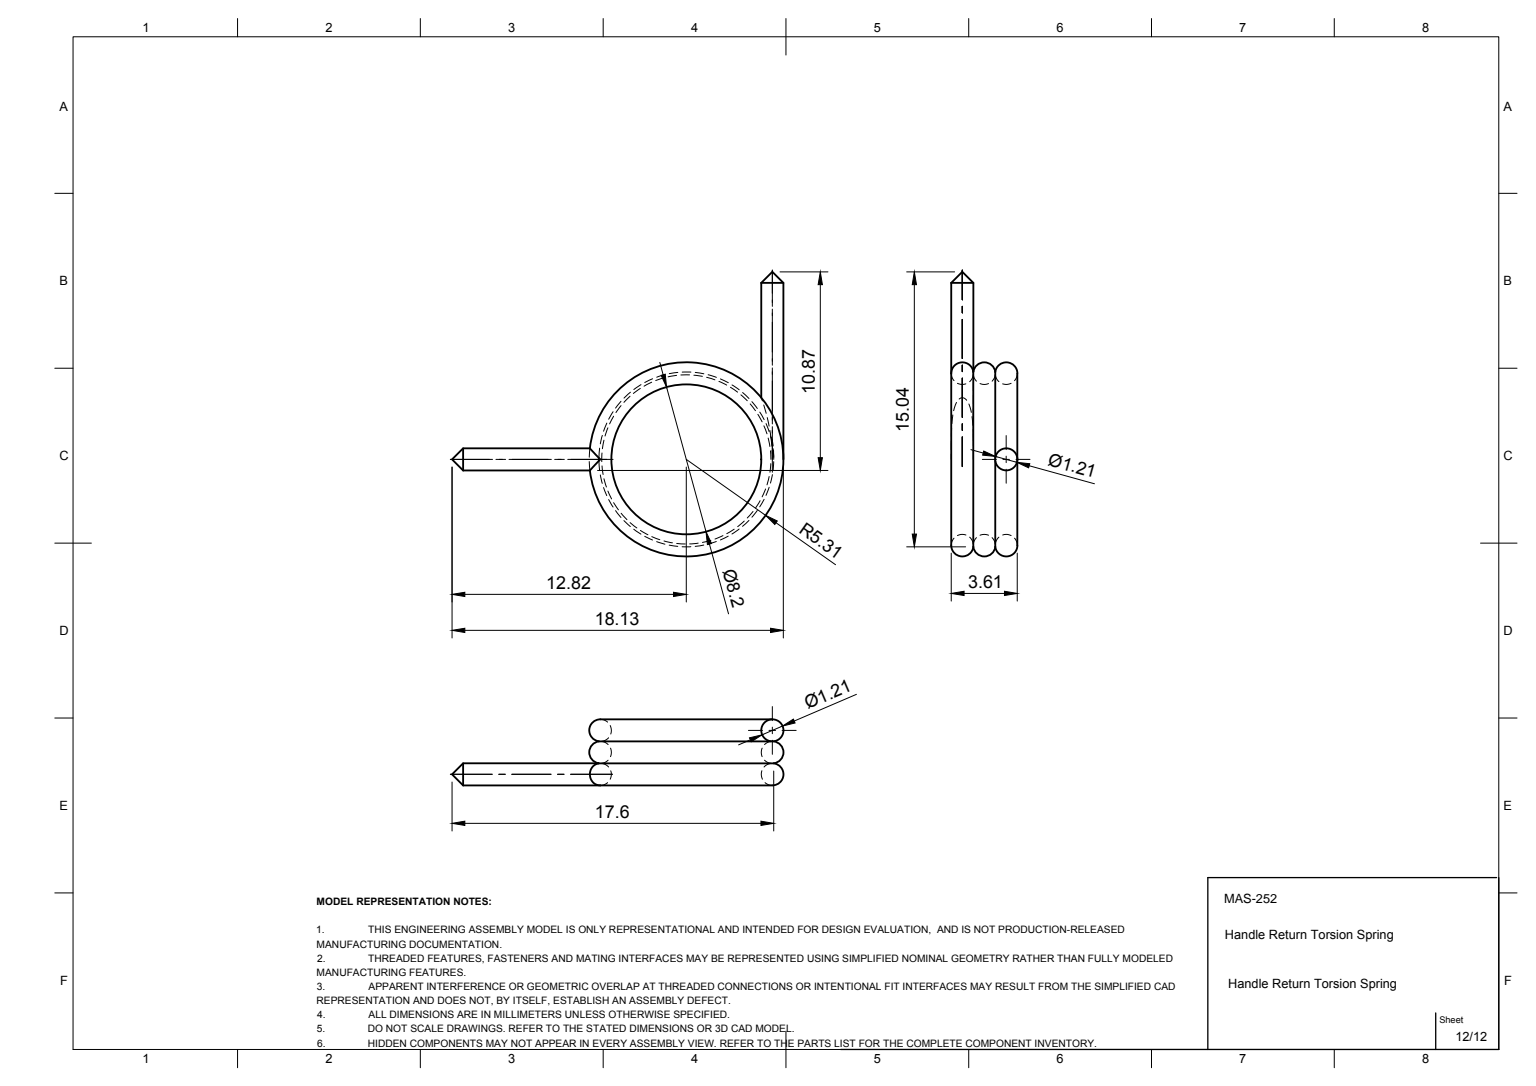
ISO-10303-21;
HEADER;
FILE_DESCRIPTION((''),'2;1');
FILE_NAME('Handle Return Torsion Spring.step','2026-10-06T07:01:46+05:00',(''),(''),'','','');
FILE_SCHEMA (('AUTOMOTIVE_DESIGN { 1 0 10303 214 3 1 1 }'));
ENDSEC;
DATA;
#10=MECHANICAL_DESIGN_GEOMETRIC_PRESENTATION_REPRESENTATION('',(#146),#11396);
#104=CONICAL_SURFACE('',#6292,0.605,0.785398163397447) ;
#105=CONICAL_SURFACE('',#6305,0.605,0.78539816339745) ;
#116=SHAPE_REPRESENTATION_RELATIONSHIP('SRR','None',#11463,#131) ;
#131=ADVANCED_BREP_SHAPE_REPRESENTATION('',(#161),#11389) ;
#146=STYLED_ITEM('',(#11547),#161) ;
#161=MANIFOLD_SOLID_BREP('Handle Return Torsion Spring',#5577) ;
#234=TOROIDAL_SURFACE('',#6293,4.705,0.605) ;
#235=TOROIDAL_SURFACE('',#6298,4.705,0.605) ;
#236=TOROIDAL_SURFACE('',#6306,4.705,0.605) ;
#237=TOROIDAL_SURFACE('',#6309,4.705,0.605) ;
#331=B_SPLINE_CURVE_WITH_KNOTS('',3,(#10992,#10993,#10994,#10995,#10996,
#10997,#10998,#10999,#11000,#11001,#11002,#11003,#11004,#11005),
 .UNSPECIFIED.,.F.,.F.,(4,2,2,2,2,2,4),(-0.0259307736234173,-0.0249485644999998,
-0.0216439933226257,-0.0192686778677155,-0.0180929024728077,-0.0172645332734243,
-0.0172587275311834),.UNSPECIFIED.) ;
#332=B_SPLINE_CURVE_WITH_KNOTS('',3,(#11007,#11008,#11009,#11010,#11011,
#11012,#11013,#11014,#11015,#11016,#11017,#11018,#11019,#11020,#11021,#11022,
#11023,#11024,#11025,#11026,#11027,#11028,#11029,#11030,#11031,#11032,#11033,
#11034),.UNSPECIFIED.,.F.,.F.,(4,2,2,2,2,2,2,2,2,2,2,2,2,4),(-0.227861047738708,
-0.227391834147561,-0.205936841126713,-0.182802806411279,-0.158511575631131,
-0.139726830403032,-0.124097041482524,-0.113695917073779,-0.103294792665033,
-0.0876650037445263,-0.0688802585164366,-0.0445890277362838,-0.0214549930208493,
-0.0104677835050617),.UNSPECIFIED.) ;
#333=B_SPLINE_CURVE_WITH_KNOTS('',3,(#11036,#11037,#11038,#11039,#11040,
#11041,#11042,#11043,#11044,#11045,#11046,#11047,#11048,#11049,#11050,#11051,
#11052,#11053,#11054,#11055,#11056,#11057,#11058,#11059,#11060,#11061,#11062,
#11063),.UNSPECIFIED.,.F.,.F.,(4,2,2,2,2,2,2,2,2,2,2,2,2,4),(-0.216924050647861,
-0.205936841131769,-0.18280280641576,-0.158511575635004,-0.139726830406447,
-0.124097041485557,-0.11369591707655,-0.103294792667543,-0.0876650037466527,
-0.0688802585180876,-0.0445890277373239,-0.0214549930213075,0.,0.000469213591169131),
 .UNSPECIFIED.) ;
#334=B_SPLINE_CURVE_WITH_KNOTS('',3,(#11064,#11065,#11066,#11067,#11068,
#11069,#11070,#11071,#11072,#11073,#11074,#11075),.UNSPECIFIED.,.F.,.F.,
(4,2,2,2,2,4),(-0.0172587275311834,-0.0164381703856616,-0.0152719978296815,
-0.0126858911745641,-0.00874619308042844,-0.00858294775784745),
 .UNSPECIFIED.) ;
#335=B_SPLINE_CURVE_WITH_KNOTS('',3,(#11092,#11093,#11094,#11095,#11096,
#11097,#11098,#11099,#11100,#11101,#11102,#11103,#11104,#11105,#11106,#11107,
#11108,#11109,#11110,#11111,#11112,#11113,#11114,#11115,#11116,#11117,#11118,
#11119),.UNSPECIFIED.,.F.,.F.,(4,2,2,2,2,2,2,2,2,2,2,2,2,4),(-0.395561282223792,
-0.371589813708337,-0.344453097699251,-0.238518055903461,-0.203039163893727,
-0.181087404891762,-0.170436776518923,-0.161871312257026,-0.152337951045022,
-0.140457204945395,-0.136918737460203,-0.135513383219719,-0.13466047941831,
-0.134248321319432),.UNSPECIFIED.) ;
#336=B_SPLINE_CURVE_WITH_KNOTS('',3,(#11126,#11127,#11128,#11129,#11130,
#11131,#11132,#11133,#11134,#11135,#11136,#11137,#11138,#11139,#11140,#11141,
#11142,#11143,#11144,#11145,#11146,#11147,#11148,#11149,#11150,#11151),
 .UNSPECIFIED.,.F.,.F.,(4,2,2,2,2,2,2,2,2,2,2,2,4),(-1.12946917222019,-0.956778050613223,
-0.699790449652219,-0.624100552674695,-0.590735740809338,-0.565825455088631,
-0.541939131211673,-0.511943639238009,-0.463169452478806,-0.380157846166964,
-0.241539556580725,0.,0.0019944793498423),.UNSPECIFIED.) ;
#797=FACE_OUTER_BOUND('',#1164,.T.) ;
#798=FACE_OUTER_BOUND('',#1165,.T.) ;
#799=FACE_OUTER_BOUND('',#1166,.T.) ;
#800=FACE_OUTER_BOUND('',#1167,.T.) ;
#801=FACE_OUTER_BOUND('',#1168,.T.) ;
#802=FACE_OUTER_BOUND('',#1169,.T.) ;
#803=FACE_OUTER_BOUND('',#1170,.T.) ;
#804=FACE_OUTER_BOUND('',#1171,.T.) ;
#1164=EDGE_LOOP('',(#4884,#4885,#4886,#4887,#4888,#4889,#4890)) ;
#1165=EDGE_LOOP('',(#4891,#4892,#4893)) ;
#1166=EDGE_LOOP('',(#4894,#4895,#4896,#4897,#4898,#4899,#4900)) ;
#1167=EDGE_LOOP('',(#4901,#4902,#4903,#4904,#4905,#4906,#4907,#4908,#4909)) ;
#1168=EDGE_LOOP('',(#4910,#4911,#4912,#4913,#4914,#4915)) ;
#1169=EDGE_LOOP('',(#4916,#4917,#4918)) ;
#1170=EDGE_LOOP('',(#4919,#4920,#4921,#4922)) ;
#1171=EDGE_LOOP('',(#4923,#4924,#4925,#4926,#4927,#4928,#4929)) ;
#1557=LINE('',#10990,#1940) ;
#1558=LINE('',#11078,#1941) ;
#1559=LINE('',#11125,#1942) ;
#1560=LINE('',#11155,#1943) ;
#1940=VECTOR('',#7835,0.605) ;
#1941=VECTOR('',#7838,0.605) ;
#1942=VECTOR('',#7861,0.605) ;
#1943=VECTOR('',#7866,0.605) ;
#2218=CIRCLE('',#6291,0.605) ;
#2219=CIRCLE('',#6294,4.6273791265187) ;
#2220=CIRCLE('',#6295,0.605) ;
#2221=CIRCLE('',#6296,4.78262087348138) ;
#2222=CIRCLE('',#6297,4.78262087348138) ;
#2223=CIRCLE('',#6299,0.605) ;
#2224=CIRCLE('',#6300,4.78262087348138) ;
#2225=CIRCLE('',#6301,4.78262087348138) ;
#2226=CIRCLE('',#6303,0.605) ;
#2227=CIRCLE('',#6304,0.605) ;
#2228=CIRCLE('',#6307,4.62737912651871) ;
#2229=CIRCLE('',#6308,0.605) ;
#2230=CIRCLE('',#6310,0.605) ;
#2677=VERTEX_POINT('',#10987) ;
#2678=VERTEX_POINT('',#10989) ;
#2679=VERTEX_POINT('',#10991) ;
#2680=VERTEX_POINT('',#11006) ;
#2681=VERTEX_POINT('',#11035) ;
#2682=VERTEX_POINT('',#11077) ;
#2683=VERTEX_POINT('',#11080) ;
#2684=VERTEX_POINT('',#11082) ;
#2685=VERTEX_POINT('',#11087) ;
#2686=VERTEX_POINT('',#11089) ;
#2687=VERTEX_POINT('',#11091) ;
#2688=VERTEX_POINT('',#11122) ;
#2689=VERTEX_POINT('',#11124) ;
#2690=VERTEX_POINT('',#11154) ;
#2691=VERTEX_POINT('',#11157) ;
#3424=EDGE_CURVE('',#2677,#2677,#2218,.T.) ;
#3425=EDGE_CURVE('',#2677,#2678,#1557,.T.) ;
#3426=EDGE_CURVE('',#2679,#2678,#331,.T.) ;
#3427=EDGE_CURVE('',#2680,#2679,#332,.T.) ;
#3428=EDGE_CURVE('',#2681,#2680,#333,.T.) ;
#3429=EDGE_CURVE('',#2678,#2681,#334,.T.) ;
#3430=EDGE_CURVE('',#2682,#2677,#1558,.T.) ;
#3431=EDGE_CURVE('',#2683,#2683,#2219,.T.) ;
#3432=EDGE_CURVE('',#2683,#2684,#2220,.T.) ;
#3433=EDGE_CURVE('',#2681,#2684,#2221,.T.) ;
#3434=EDGE_CURVE('',#2684,#2679,#2222,.T.) ;
#3435=EDGE_CURVE('',#2684,#2685,#2223,.T.) ;
#3436=EDGE_CURVE('',#2686,#2685,#2224,.T.) ;
#3437=EDGE_CURVE('',#2686,#2687,#335,.T.) ;
#3438=EDGE_CURVE('',#2685,#2687,#2225,.T.) ;
#3439=EDGE_CURVE('',#2688,#2688,#2226,.T.) ;
#3440=EDGE_CURVE('',#2688,#2689,#1559,.T.) ;
#3441=EDGE_CURVE('',#2687,#2689,#336,.T.) ;
#3442=EDGE_CURVE('',#2689,#2686,#2227,.T.) ;
#3443=EDGE_CURVE('',#2690,#2688,#1560,.T.) ;
#3444=EDGE_CURVE('',#2691,#2691,#2228,.T.) ;
#3445=EDGE_CURVE('',#2691,#2683,#2229,.T.) ;
#3446=EDGE_CURVE('',#2685,#2691,#2230,.T.) ;
#4884=ORIENTED_EDGE('',*,*,#3424,.F.) ;
#4885=ORIENTED_EDGE('',*,*,#3425,.T.) ;
#4886=ORIENTED_EDGE('',*,*,#3426,.F.) ;
#4887=ORIENTED_EDGE('',*,*,#3427,.F.) ;
#4888=ORIENTED_EDGE('',*,*,#3428,.F.) ;
#4889=ORIENTED_EDGE('',*,*,#3429,.F.) ;
#4890=ORIENTED_EDGE('',*,*,#3425,.F.) ;
#4891=ORIENTED_EDGE('',*,*,#3430,.T.) ;
#4892=ORIENTED_EDGE('',*,*,#3424,.T.) ;
#4893=ORIENTED_EDGE('',*,*,#3430,.F.) ;
#4894=ORIENTED_EDGE('',*,*,#3431,.F.) ;
#4895=ORIENTED_EDGE('',*,*,#3432,.T.) ;
#4896=ORIENTED_EDGE('',*,*,#3433,.F.) ;
#4897=ORIENTED_EDGE('',*,*,#3428,.T.) ;
#4898=ORIENTED_EDGE('',*,*,#3427,.T.) ;
#4899=ORIENTED_EDGE('',*,*,#3434,.F.) ;
#4900=ORIENTED_EDGE('',*,*,#3432,.F.) ;
#4901=ORIENTED_EDGE('',*,*,#3426,.T.) ;
#4902=ORIENTED_EDGE('',*,*,#3429,.T.) ;
#4903=ORIENTED_EDGE('',*,*,#3433,.T.) ;
#4904=ORIENTED_EDGE('',*,*,#3435,.T.) ;
#4905=ORIENTED_EDGE('',*,*,#3436,.F.) ;
#4906=ORIENTED_EDGE('',*,*,#3437,.T.) ;
#4907=ORIENTED_EDGE('',*,*,#3438,.F.) ;
#4908=ORIENTED_EDGE('',*,*,#3435,.F.) ;
#4909=ORIENTED_EDGE('',*,*,#3434,.T.) ;
#4910=ORIENTED_EDGE('',*,*,#3439,.F.) ;
#4911=ORIENTED_EDGE('',*,*,#3440,.T.) ;
#4912=ORIENTED_EDGE('',*,*,#3441,.F.) ;
#4913=ORIENTED_EDGE('',*,*,#3437,.F.) ;
#4914=ORIENTED_EDGE('',*,*,#3442,.F.) ;
#4915=ORIENTED_EDGE('',*,*,#3440,.F.) ;
#4916=ORIENTED_EDGE('',*,*,#3443,.T.) ;
#4917=ORIENTED_EDGE('',*,*,#3439,.T.) ;
#4918=ORIENTED_EDGE('',*,*,#3443,.F.) ;
#4919=ORIENTED_EDGE('',*,*,#3444,.F.) ;
#4920=ORIENTED_EDGE('',*,*,#3445,.T.) ;
#4921=ORIENTED_EDGE('',*,*,#3431,.T.) ;
#4922=ORIENTED_EDGE('',*,*,#3445,.F.) ;
#4923=ORIENTED_EDGE('',*,*,#3442,.T.) ;
#4924=ORIENTED_EDGE('',*,*,#3436,.T.) ;
#4925=ORIENTED_EDGE('',*,*,#3446,.T.) ;
#4926=ORIENTED_EDGE('',*,*,#3444,.T.) ;
#4927=ORIENTED_EDGE('',*,*,#3446,.F.) ;
#4928=ORIENTED_EDGE('',*,*,#3438,.T.) ;
#4929=ORIENTED_EDGE('',*,*,#3441,.T.) ;
#5212=CYLINDRICAL_SURFACE('',#6290,0.605) ;
#5213=CYLINDRICAL_SURFACE('',#6302,0.605) ;
#5522=ADVANCED_FACE('',(#797),#5212,.T.) ;
#5523=ADVANCED_FACE('',(#798),#104,.T.) ;
#5524=ADVANCED_FACE('',(#799),#234,.T.) ;
#5525=ADVANCED_FACE('',(#800),#235,.T.) ;
#5526=ADVANCED_FACE('',(#801),#5213,.T.) ;
#5527=ADVANCED_FACE('',(#802),#105,.T.) ;
#5528=ADVANCED_FACE('',(#803),#236,.T.) ;
#5529=ADVANCED_FACE('',(#804),#237,.T.) ;
#5577=CLOSED_SHELL('',(#5522,#5523,#5524,#5525,#5526,#5527,#5528,#5529)) ;
#6289=AXIS2_PLACEMENT_3D('',#10985,#7829,#7830) ;
#6290=AXIS2_PLACEMENT_3D('',#10986,#7831,#7832) ;
#6291=AXIS2_PLACEMENT_3D('',#10988,#7833,#7834) ;
#6292=AXIS2_PLACEMENT_3D('',#11076,#7836,#7837) ;
#6293=AXIS2_PLACEMENT_3D('',#11079,#7839,#7840) ;
#6294=AXIS2_PLACEMENT_3D('',#11081,#7841,#7842) ;
#6295=AXIS2_PLACEMENT_3D('',#11083,#7843,#7844) ;
#6296=AXIS2_PLACEMENT_3D('',#11084,#7845,#7846) ;
#6297=AXIS2_PLACEMENT_3D('',#11085,#7847,#7848) ;
#6298=AXIS2_PLACEMENT_3D('',#11086,#7849,#7850) ;
#6299=AXIS2_PLACEMENT_3D('',#11088,#7851,#7852) ;
#6300=AXIS2_PLACEMENT_3D('',#11090,#7853,#7854) ;
#6301=AXIS2_PLACEMENT_3D('',#11120,#7855,#7856) ;
#6302=AXIS2_PLACEMENT_3D('',#11121,#7857,#7858) ;
#6303=AXIS2_PLACEMENT_3D('',#11123,#7859,#7860) ;
#6304=AXIS2_PLACEMENT_3D('',#11152,#7862,#7863) ;
#6305=AXIS2_PLACEMENT_3D('',#11153,#7864,#7865) ;
#6306=AXIS2_PLACEMENT_3D('',#11156,#7867,#7868) ;
#6307=AXIS2_PLACEMENT_3D('',#11158,#7869,#7870) ;
#6308=AXIS2_PLACEMENT_3D('',#11159,#7871,#7872) ;
#6309=AXIS2_PLACEMENT_3D('',#11160,#7873,#7874) ;
#6310=AXIS2_PLACEMENT_3D('',#11161,#7875,#7876) ;
#7829=DIRECTION('axis',(0.,0.,1.)) ;
#7830=DIRECTION('refdir',(1.,0.,0.)) ;
#7831=DIRECTION('center_axis',(0.,-1.,0.)) ;
#7832=DIRECTION('ref_axis',(1.,0.,0.)) ;
#7833=DIRECTION('center_axis',(0.,-1.,0.)) ;
#7834=DIRECTION('ref_axis',(1.,0.,0.)) ;
#7835=DIRECTION('',(0.,1.,0.)) ;
#7836=DIRECTION('center_axis',(0.,1.,0.)) ;
#7837=DIRECTION('ref_axis',(1.,0.,0.)) ;
#7838=DIRECTION('',(-0.707106781186547,0.707106781186548,-8.65956056235493E-17)) ;
#7839=DIRECTION('center_axis',(1.,0.,0.)) ;
#7840=DIRECTION('ref_axis',(0.,0.,-1.)) ;
#7841=DIRECTION('center_axis',(1.,0.,0.)) ;
#7842=DIRECTION('ref_axis',(0.,0.,-1.)) ;
#7843=DIRECTION('center_axis',(0.,-1.,0.)) ;
#7844=DIRECTION('ref_axis',(0.,0.,1.)) ;
#7845=DIRECTION('center_axis',(-1.,0.,0.)) ;
#7846=DIRECTION('ref_axis',(0.,-4.6427390085679E-16,-1.)) ;
#7847=DIRECTION('center_axis',(-1.,0.,0.)) ;
#7848=DIRECTION('ref_axis',(0.,-4.6427390085679E-16,-1.)) ;
#7849=DIRECTION('center_axis',(1.,0.,0.)) ;
#7850=DIRECTION('ref_axis',(0.,0.,-1.)) ;
#7851=DIRECTION('center_axis',(0.,-1.,0.)) ;
#7852=DIRECTION('ref_axis',(0.,0.,1.)) ;
#7853=DIRECTION('center_axis',(-1.,0.,0.)) ;
#7854=DIRECTION('ref_axis',(0.,0.,-1.)) ;
#7855=DIRECTION('center_axis',(-1.,0.,0.)) ;
#7856=DIRECTION('ref_axis',(0.,0.,-1.)) ;
#7857=DIRECTION('center_axis',(0.,0.,1.)) ;
#7858=DIRECTION('ref_axis',(1.,0.,0.)) ;
#7859=DIRECTION('center_axis',(0.,0.,1.)) ;
#7860=DIRECTION('ref_axis',(1.,0.,0.)) ;
#7861=DIRECTION('',(0.,0.,-1.)) ;
#7862=DIRECTION('center_axis',(0.,0.,-1.)) ;
#7863=DIRECTION('ref_axis',(0.,1.,0.)) ;
#7864=DIRECTION('center_axis',(0.,0.,-1.)) ;
#7865=DIRECTION('ref_axis',(1.,0.,0.)) ;
#7866=DIRECTION('',(-0.707106781186549,-8.65956056235495E-17,-0.707106781186546)) ;
#7867=DIRECTION('center_axis',(1.,0.,0.)) ;
#7868=DIRECTION('ref_axis',(0.,0.,-1.)) ;
#7869=DIRECTION('center_axis',(1.,0.,0.)) ;
#7870=DIRECTION('ref_axis',(0.,0.,-1.)) ;
#7871=DIRECTION('center_axis',(0.,-1.,0.)) ;
#7872=DIRECTION('ref_axis',(0.,0.,1.)) ;
#7873=DIRECTION('center_axis',(1.,0.,0.)) ;
#7874=DIRECTION('ref_axis',(0.,0.,-1.)) ;
#7875=DIRECTION('center_axis',(0.,-1.,0.)) ;
#7876=DIRECTION('ref_axis',(0.,0.,1.)) ;
#10985=CARTESIAN_POINT('',(0.,0.,0.)) ;
#10986=CARTESIAN_POINT('Origin',(-11.75,9.1075,27.14)) ;
#10987=CARTESIAN_POINT('',(-12.355,5.355,27.14)) ;
#10988=CARTESIAN_POINT('Origin',(-11.75,5.355,27.14)) ;
#10989=CARTESIAN_POINT('',(-12.355,12.750455488499,27.14)) ;
#10990=CARTESIAN_POINT('',(-12.355,9.1075,27.14)) ;
#10991=CARTESIAN_POINT('',(-12.35,12.7830090527627,27.0623791265186)) ;
#10992=CARTESIAN_POINT('Ctrl Pts',(-12.35,12.7830090527627,27.0623791265187)) ;
#10993=CARTESIAN_POINT('Ctrl Pts',(-12.3502950737228,12.7806908448569,27.0646600108443)) ;
#10994=CARTESIAN_POINT('Ctrl Pts',(-12.3505904901271,12.7784722155657,27.0670457451062)) ;
#10995=CARTESIAN_POINT('Ctrl Pts',(-12.351862421125,12.7692567705477,27.0778913302007)) ;
#10996=CARTESIAN_POINT('Ctrl Pts',(-12.3527834432199,12.7634507316376,27.0872752238927)) ;
#10997=CARTESIAN_POINT('Ctrl Pts',(-12.3540107602705,12.7560509464893,27.1046573139882)) ;
#10998=CARTESIAN_POINT('Ctrl Pts',(-12.3544131665346,12.7537562758761,27.1122458244381)) ;
#10999=CARTESIAN_POINT('Ctrl Pts',(-12.3547973310216,12.7515851944735,27.1238745715472)) ;
#11000=CARTESIAN_POINT('Ctrl Pts',(-12.35488882304,12.7510746489759,27.1277615519975)) ;
#11001=CARTESIAN_POINT('Ctrl Pts',(-12.3549805414859,12.7505634754885,27.1344212175193)) ;
#11002=CARTESIAN_POINT('Ctrl Pts',(-12.354999732288,12.7504569762397,27.1371809648499)) ;
#11003=CARTESIAN_POINT('Ctrl Pts',(-12.3549999990716,12.7504554936582,27.1399612986886)) ;
#11004=CARTESIAN_POINT('Ctrl Pts',(-12.355,12.750455488499,27.1399806493727)) ;
#11005=CARTESIAN_POINT('Ctrl Pts',(-12.355,12.750455488499,27.14)) ;
#11006=CARTESIAN_POINT('',(-11.145,12.86,27.14)) ;
#11007=CARTESIAN_POINT('Ctrl Pts',(-11.145,12.86,27.14)) ;
#11008=CARTESIAN_POINT('Ctrl Pts',(-11.145,12.8588940529596,27.1388940529596)) ;
#11009=CARTESIAN_POINT('Ctrl Pts',(-11.1450030325259,12.8577882989711,27.1377879090259)) ;
#11010=CARTESIAN_POINT('Ctrl Pts',(-11.1452865760822,12.8061310509855,27.0860942402119)) ;
#11011=CARTESIAN_POINT('Ctrl Pts',(-11.1519114742386,12.7558318101249,27.0349322751955)) ;
#11012=CARTESIAN_POINT('Ctrl Pts',(-11.1797923903892,12.6543074731248,26.9301061021828)) ;
#11013=CARTESIAN_POINT('Ctrl Pts',(-11.2022679712777,12.602916384759,26.8761391748599)) ;
#11014=CARTESIAN_POINT('Ctrl Pts',(-11.2664077022682,12.504207481754,26.771026596332)) ;
#11015=CARTESIAN_POINT('Ctrl Pts',(-11.3092184518965,12.4568810929982,26.7197878129444)) ;
#11016=CARTESIAN_POINT('Ctrl Pts',(-11.404006903276,12.3846941955802,26.6407914702403)) ;
#11017=CARTESIAN_POINT('Ctrl Pts',(-11.4515986829293,12.3572803837341,26.6104713174002)) ;
#11018=CARTESIAN_POINT('Ctrl Pts',(-11.5495504041745,12.318257424657,26.567102172624)) ;
#11019=CARTESIAN_POINT('Ctrl Pts',(-11.597430122757,12.3050452142842,26.552323078106)) ;
#11020=CARTESIAN_POINT('Ctrl Pts',(-11.6814023169578,12.2921970431839,26.5379383989027)) ;
#11021=CARTESIAN_POINT('Ctrl Pts',(-11.7155770857141,12.2895782159149,26.535)) ;
#11022=CARTESIAN_POINT('Ctrl Pts',(-11.7844229142859,12.2895782159149,26.535)) ;
#11023=CARTESIAN_POINT('Ctrl Pts',(-11.8185976830422,12.2921970431839,26.5379383989027)) ;
#11024=CARTESIAN_POINT('Ctrl Pts',(-11.902569877243,12.3050452142842,26.552323078106)) ;
#11025=CARTESIAN_POINT('Ctrl Pts',(-11.9504495958255,12.318257424657,26.567102172624)) ;
#11026=CARTESIAN_POINT('Ctrl Pts',(-12.0484013170707,12.3572803837341,26.6104713174002)) ;
#11027=CARTESIAN_POINT('Ctrl Pts',(-12.095993096724,12.3846941955802,26.6407914702403)) ;
#11028=CARTESIAN_POINT('Ctrl Pts',(-12.1907815481035,12.4568810929982,26.7197878129444)) ;
#11029=CARTESIAN_POINT('Ctrl Pts',(-12.2335922977317,12.504207481754,26.771026596332)) ;
#11030=CARTESIAN_POINT('Ctrl Pts',(-12.2977320287223,12.602916384759,26.8761391748599)) ;
#11031=CARTESIAN_POINT('Ctrl Pts',(-12.3202076096108,12.6543074731248,26.9301061021828)) ;
#11032=CARTESIAN_POINT('Ctrl Pts',(-12.3415431622717,12.7319978125214,27.0103231338782)) ;
#11033=CARTESIAN_POINT('Ctrl Pts',(-12.3466318999977,12.7573932140223,27.0363441193002)) ;
#11034=CARTESIAN_POINT('Ctrl Pts',(-12.35,12.7830090527627,27.0623791265186)) ;
#11035=CARTESIAN_POINT('',(-12.35,12.7830090527627,27.2176208734814)) ;
#11036=CARTESIAN_POINT('Ctrl Pts',(-12.35,12.7830090527627,27.2176208734814)) ;
#11037=CARTESIAN_POINT('Ctrl Pts',(-12.3466318999977,12.7573932140222,27.2436558806998)) ;
#11038=CARTESIAN_POINT('Ctrl Pts',(-12.3415431622717,12.7319978125214,27.2696768661217)) ;
#11039=CARTESIAN_POINT('Ctrl Pts',(-12.3202076096108,12.6543074731248,27.3498938978172)) ;
#11040=CARTESIAN_POINT('Ctrl Pts',(-12.2977320287223,12.602916384759,27.4038608251401)) ;
#11041=CARTESIAN_POINT('Ctrl Pts',(-12.2335922977317,12.504207481754,27.508973403668)) ;
#11042=CARTESIAN_POINT('Ctrl Pts',(-12.1907815481035,12.4568810929982,27.5602121870556)) ;
#11043=CARTESIAN_POINT('Ctrl Pts',(-12.095993096724,12.3846941955802,27.6392085297597)) ;
#11044=CARTESIAN_POINT('Ctrl Pts',(-12.0484013170707,12.3572803837341,27.6695286825999)) ;
#11045=CARTESIAN_POINT('Ctrl Pts',(-11.9504495958255,12.318257424657,27.712897827376)) ;
#11046=CARTESIAN_POINT('Ctrl Pts',(-11.902569877243,12.3050452142842,27.727676921894)) ;
#11047=CARTESIAN_POINT('Ctrl Pts',(-11.8185976830421,12.2921970431839,27.7420616010973)) ;
#11048=CARTESIAN_POINT('Ctrl Pts',(-11.7844229142859,12.2895782159149,27.745)) ;
#11049=CARTESIAN_POINT('Ctrl Pts',(-11.7155770857141,12.2895782159149,27.745)) ;
#11050=CARTESIAN_POINT('Ctrl Pts',(-11.6814023169579,12.2921970431839,27.7420616010973)) ;
#11051=CARTESIAN_POINT('Ctrl Pts',(-11.597430122757,12.3050452142842,27.727676921894)) ;
#11052=CARTESIAN_POINT('Ctrl Pts',(-11.5495504041744,12.318257424657,27.712897827376)) ;
#11053=CARTESIAN_POINT('Ctrl Pts',(-11.4515986829293,12.3572803837341,27.6695286825999)) ;
#11054=CARTESIAN_POINT('Ctrl Pts',(-11.404006903276,12.3846941955802,27.6392085297597)) ;
#11055=CARTESIAN_POINT('Ctrl Pts',(-11.3092184518965,12.4568810929982,27.5602121870556)) ;
#11056=CARTESIAN_POINT('Ctrl Pts',(-11.2664077022683,12.504207481754,27.508973403668)) ;
#11057=CARTESIAN_POINT('Ctrl Pts',(-11.2022679712777,12.602916384759,27.4038608251401)) ;
#11058=CARTESIAN_POINT('Ctrl Pts',(-11.1797923903892,12.6543074731248,27.3498938978172)) ;
#11059=CARTESIAN_POINT('Ctrl Pts',(-11.1519114742386,12.7558318101248,27.2450677248047)) ;
#11060=CARTESIAN_POINT('Ctrl Pts',(-11.1452865760822,12.8061310509845,27.1939057597892)) ;
#11061=CARTESIAN_POINT('Ctrl Pts',(-11.1450030325259,12.8577882989711,27.142212090974)) ;
#11062=CARTESIAN_POINT('Ctrl Pts',(-11.145,12.8588940529595,27.1411059470405)) ;
#11063=CARTESIAN_POINT('Ctrl Pts',(-11.145,12.86,27.14)) ;
#11064=CARTESIAN_POINT('Ctrl Pts',(-12.355,12.750455488499,27.14)) ;
#11065=CARTESIAN_POINT('Ctrl Pts',(-12.355,12.750455488499,27.1427349294549)) ;
#11066=CARTESIAN_POINT('Ctrl Pts',(-12.3549814299797,12.7505585433804,27.1454687221292)) ;
#11067=CARTESIAN_POINT('Ctrl Pts',(-12.3548919814718,12.7510570192555,27.1520711674936)) ;
#11068=CARTESIAN_POINT('Ctrl Pts',(-12.3548023926968,12.7515568704589,27.1559272391055)) ;
#11069=CARTESIAN_POINT('Ctrl Pts',(-12.354400939583,12.7538247773979,27.1682198224544)) ;
#11070=CARTESIAN_POINT('Ctrl Pts',(-12.3539513532903,12.7563863566276,27.1764662136017)) ;
#11071=CARTESIAN_POINT('Ctrl Pts',(-12.3524955292764,12.7652281510509,27.1962856643817)) ;
#11072=CARTESIAN_POINT('Ctrl Pts',(-12.3513337250394,12.7726732154684,27.2071627127485)) ;
#11073=CARTESIAN_POINT('Ctrl Pts',(-12.3500982949853,12.7822396470076,27.2168582304118)) ;
#11074=CARTESIAN_POINT('Ctrl Pts',(-12.3500491385241,12.7826230024089,27.2172410386102)) ;
#11075=CARTESIAN_POINT('Ctrl Pts',(-12.35,12.7830090527627,27.2176208734813)) ;
#11076=CARTESIAN_POINT('Origin',(-11.75,5.355,27.14)) ;
#11077=CARTESIAN_POINT('',(-11.75,4.75,27.14)) ;
#11078=CARTESIAN_POINT('',(-12.355,5.355,27.14)) ;
#11079=CARTESIAN_POINT('Origin',(-11.75,17.565,27.14)) ;
#11080=CARTESIAN_POINT('',(-12.35,17.565,31.7673791265187)) ;
#11081=CARTESIAN_POINT('Origin',(-12.35,17.565,27.14)) ;
#11082=CARTESIAN_POINT('',(-12.35,17.565,31.9226208734814)) ;
#11083=CARTESIAN_POINT('Origin',(-11.75,17.565,31.845)) ;
#11084=CARTESIAN_POINT('Origin',(-12.35,17.565,27.14)) ;
#11085=CARTESIAN_POINT('Origin',(-12.35,17.565,27.14)) ;
#11086=CARTESIAN_POINT('Origin',(-12.95,17.565,27.14)) ;
#11087=CARTESIAN_POINT('',(-13.55,17.565,31.9226208734814)) ;
#11088=CARTESIAN_POINT('Origin',(-12.95,17.565,31.845)) ;
#11089=CARTESIAN_POINT('',(-13.55,22.3476208734813,27.14)) ;
#11090=CARTESIAN_POINT('Origin',(-13.55,17.565,27.14)) ;
#11091=CARTESIAN_POINT('',(-13.55,22.1923791265188,28.348645869938)) ;
#11092=CARTESIAN_POINT('Ctrl Pts',(-13.55,22.3476208734813,27.14)) ;
#11093=CARTESIAN_POINT('Ctrl Pts',(-13.55,22.3476208734813,27.1768198202397)) ;
#11094=CARTESIAN_POINT('Ctrl Pts',(-13.549972380845,22.3474082907238,27.2137523858758)) ;
#11095=CARTESIAN_POINT('Ctrl Pts',(-13.5498550016055,22.3464932731043,27.2922511809408)) ;
#11096=CARTESIAN_POINT('Ctrl Pts',(-13.5497569884623,22.345726361199,27.334087768373)) ;
#11097=CARTESIAN_POINT('Ctrl Pts',(-13.5491067207649,22.3404972586508,27.5384500571714)) ;
#11098=CARTESIAN_POINT('Ctrl Pts',(-13.5478768740312,22.3314507737802,27.7118712318312)) ;
#11099=CARTESIAN_POINT('Ctrl Pts',(-13.54618269997,22.3082584061997,27.9279108422923)) ;
#11100=CARTESIAN_POINT('Ctrl Pts',(-13.5457497913871,22.3012634140032,27.9830733402867)) ;
#11101=CARTESIAN_POINT('Ctrl Pts',(-13.5452354453862,22.2876608351609,28.0701147047968)) ;
#11102=CARTESIAN_POINT('Ctrl Pts',(-13.5450774384555,22.2817529911622,28.1039281404144)) ;
#11103=CARTESIAN_POINT('Ctrl Pts',(-13.5449941917603,22.2718528068373,28.1528901788853)) ;
#11104=CARTESIAN_POINT('Ctrl Pts',(-13.5449907726018,22.2683775902305,28.1689937520493)) ;
#11105=CARTESIAN_POINT('Ctrl Pts',(-13.5450498894599,22.2616760847522,28.1976545310589)) ;
#11106=CARTESIAN_POINT('Ctrl Pts',(-13.5451001605247,22.2584789754413,28.2105249581503)) ;
#11107=CARTESIAN_POINT('Ctrl Pts',(-13.5452772351488,22.2513001281173,28.2372934647939)) ;
#11108=CARTESIAN_POINT('Ctrl Pts',(-13.5454156907078,22.2471245647707,28.2516872843723)) ;
#11109=CARTESIAN_POINT('Ctrl Pts',(-13.5458759084847,22.236971562035,28.2828399779785)) ;
#11110=CARTESIAN_POINT('Ctrl Pts',(-13.5463763020817,22.2278127187268,28.3085246705737)) ;
#11111=CARTESIAN_POINT('Ctrl Pts',(-13.5476010192359,22.2138681250654,28.3323856779711)) ;
#11112=CARTESIAN_POINT('Ctrl Pts',(-13.5479924036389,22.2097234593898,28.3385876920861)) ;
#11113=CARTESIAN_POINT('Ctrl Pts',(-13.5486856107791,22.2032963110619,28.3447037146101)) ;
#11114=CARTESIAN_POINT('Ctrl Pts',(-13.5489212711138,22.2011915586321,28.3463515782256)) ;
#11115=CARTESIAN_POINT('Ctrl Pts',(-13.5493534389941,22.1975387087175,28.3480922560446)) ;
#11116=CARTESIAN_POINT('Ctrl Pts',(-13.5495314705389,22.1960751072108,28.3485524698715)) ;
#11117=CARTESIAN_POINT('Ctrl Pts',(-13.5498146884684,22.1938216608994,28.348751241983)) ;
#11118=CARTESIAN_POINT('Ctrl Pts',(-13.5499072651155,22.193095956003,28.3487379414572)) ;
#11119=CARTESIAN_POINT('Ctrl Pts',(-13.55,22.1923791265188,28.348645869938)) ;
#11120=CARTESIAN_POINT('Origin',(-13.55,17.565,27.14)) ;
#11121=CARTESIAN_POINT('Origin',(-14.15,22.27,31.9675)) ;
#11122=CARTESIAN_POINT('',(-14.755,22.27,36.795)) ;
#11123=CARTESIAN_POINT('Origin',(-14.15,22.27,36.795)) ;
#11124=CARTESIAN_POINT('',(-14.755,22.27,27.14)) ;
#11125=CARTESIAN_POINT('',(-14.755,22.27,31.9675)) ;
#11126=CARTESIAN_POINT('Ctrl Pts',(-13.55,22.1923791265187,28.348645869938)) ;
#11127=CARTESIAN_POINT('Ctrl Pts',(-13.555980959365,22.1461470312326,28.708589197808)) ;
#11128=CARTESIAN_POINT('Ctrl Pts',(-13.5697274043909,22.0836295573281,29.0348924571245)) ;
#11129=CARTESIAN_POINT('Ctrl Pts',(-13.6464455195548,21.917193693991,29.7522595939977)) ;
#11130=CARTESIAN_POINT('Ctrl Pts',(-13.7272582418671,21.8188959714164,30.0605199827462)) ;
#11131=CARTESIAN_POINT('Ctrl Pts',(-13.8680079875454,21.7334283833394,30.3183200144738)) ;
#11132=CARTESIAN_POINT('Ctrl Pts',(-13.9166610257102,21.7077100487269,30.3934861511264)) ;
#11133=CARTESIAN_POINT('Ctrl Pts',(-14.0104457744483,21.6805579624522,30.470744338011)) ;
#11134=CARTESIAN_POINT('Ctrl Pts',(-14.042911122621,21.6734580642535,30.4906806551043)) ;
#11135=CARTESIAN_POINT('Ctrl Pts',(-14.105575612671,21.6660305679511,30.5114660985244)) ;
#11136=CARTESIAN_POINT('Ctrl Pts',(-14.133277320298,21.6645670989146,30.5155369209607)) ;
#11137=CARTESIAN_POINT('Ctrl Pts',(-14.1887990687983,21.6656337479518,30.5125620801082)) ;
#11138=CARTESIAN_POINT('Ctrl Pts',(-14.2149355044828,21.6679695920752,30.5060543395646)) ;
#11139=CARTESIAN_POINT('Ctrl Pts',(-14.2710265332359,21.6763885397882,30.4824452752556)) ;
#11140=CARTESIAN_POINT('Ctrl Pts',(-14.299405737975,21.6831426050256,30.4634213485577)) ;
#11141=CARTESIAN_POINT('Ctrl Pts',(-14.3658614796489,21.7031877288451,30.4062912197373)) ;
#11142=CARTESIAN_POINT('Ctrl Pts',(-14.400924765314,21.7185093863992,30.361968959399)) ;
#11143=CARTESIAN_POINT('Ctrl Pts',(-14.4796386580391,21.7596156952845,30.2402120334489)) ;
#11144=CARTESIAN_POINT('Ctrl Pts',(-14.525444852263,21.7923656038144,30.1407640089788)) ;
#11145=CARTESIAN_POINT('Ctrl Pts',(-14.632899615836,21.8939824451754,29.8083114879267)) ;
#11146=CARTESIAN_POINT('Ctrl Pts',(-14.6800182275857,21.9682867232431,29.5444972259161)) ;
#11147=CARTESIAN_POINT('Ctrl Pts',(-14.7604629666096,22.163462031111,28.662786627042)) ;
#11148=CARTESIAN_POINT('Ctrl Pts',(-14.7549999400109,22.2682723645561,27.965074853559)) ;
#11149=CARTESIAN_POINT('Ctrl Pts',(-14.7550000001231,22.2699929543206,27.1532965572106)) ;
#11150=CARTESIAN_POINT('Ctrl Pts',(-14.755,22.27,27.1466482644995)) ;
#11151=CARTESIAN_POINT('Ctrl Pts',(-14.755,22.27,27.14)) ;
#11152=CARTESIAN_POINT('Origin',(-14.15,22.27,27.14)) ;
#11153=CARTESIAN_POINT('Origin',(-14.15,22.27,36.795)) ;
#11154=CARTESIAN_POINT('',(-14.15,22.27,37.4)) ;
#11155=CARTESIAN_POINT('',(-14.755,22.27,36.795)) ;
#11156=CARTESIAN_POINT('Origin',(-12.95,17.565,27.14)) ;
#11157=CARTESIAN_POINT('',(-13.55,17.565,31.7673791265187)) ;
#11158=CARTESIAN_POINT('Origin',(-13.55,17.565,27.14)) ;
#11159=CARTESIAN_POINT('Origin',(-12.95,17.565,31.845)) ;
#11160=CARTESIAN_POINT('Origin',(-14.15,17.565,27.14)) ;
#11161=CARTESIAN_POINT('Origin',(-14.15,17.565,31.845)) ;
#11372=UNCERTAINTY_MEASURE_WITH_UNIT(LENGTH_MEASURE(0.01),#11397,
'DISTANCE_ACCURACY_VALUE',
'Maximum model space distance between geometric entities at asserted c
onnectivities') ;
#11379=UNCERTAINTY_MEASURE_WITH_UNIT(LENGTH_MEASURE(0.01),#11397,
'DISTANCE_ACCURACY_VALUE',
'Maximum model space distance between geometric entities at asserted c
onnectivities') ;
#11389=(
GEOMETRIC_REPRESENTATION_CONTEXT(3)
GLOBAL_UNCERTAINTY_ASSIGNED_CONTEXT((#11372))
GLOBAL_UNIT_ASSIGNED_CONTEXT((#11397,#11399,#11400))
REPRESENTATION_CONTEXT('','3D')
) ;
#11396=(
GEOMETRIC_REPRESENTATION_CONTEXT(3)
GLOBAL_UNCERTAINTY_ASSIGNED_CONTEXT((#11379))
GLOBAL_UNIT_ASSIGNED_CONTEXT((#11397,#11399,#11400))
REPRESENTATION_CONTEXT('','3D')
) ;
#11397=(
LENGTH_UNIT()
NAMED_UNIT(*)
SI_UNIT(.MILLI.,.METRE.)
) ;
#11399=(
NAMED_UNIT(*)
PLANE_ANGLE_UNIT()
SI_UNIT($,.RADIAN.)
) ;
#11400=(
NAMED_UNIT(*)
SI_UNIT($,.STERADIAN.)
SOLID_ANGLE_UNIT()
) ;
#11410=SHAPE_DEFINITION_REPRESENTATION(#11426,#11463) ;
#11426=PRODUCT_DEFINITION_SHAPE('',$,#11480) ;
#11463=SHAPE_REPRESENTATION('',(#6289),#11389) ;
#11470=PRODUCT_DEFINITION_CONTEXT('part definition',#11520,'design') ;
#11480=PRODUCT_DEFINITION('Handle Return Torsion Spring',
'Handle Return Torsion Spring',#11496,#11470) ;
#11496=PRODUCT_DEFINITION_FORMATION('',$,#11531) ;
#11520=APPLICATION_CONTEXT(
'Core Data for Automotive Mechanical Design Process') ;
#11521=PRODUCT_CONTEXT('part definition',#11520,'mechanical') ;
#11531=PRODUCT('Handle Return Torsion Spring','Handle Return Torsion Spring',
$,(#11521)) ;
#11547=PRESENTATION_STYLE_ASSIGNMENT((#11563)) ;
#11563=SURFACE_STYLE_USAGE(.BOTH.,#11579) ;
#11579=SURFACE_SIDE_STYLE('',(#11595)) ;
#11595=SURFACE_STYLE_FILL_AREA(#11611) ;
#11611=FILL_AREA_STYLE(
'MAS-252 Metallic - Handle Return Torsion Spring',(#11627)) ;
#11627=FILL_AREA_STYLE_COLOUR(
'MAS-252 Metallic - Handle Return Torsion Spring',#11643) ;
#11643=COLOUR_RGB('MAS-252 Metallic - Handle Return Torsion Spring', 0.31764706, 0.68627451, 0.89019608) ;
ENDSEC;
END-ISO-10303-21;
